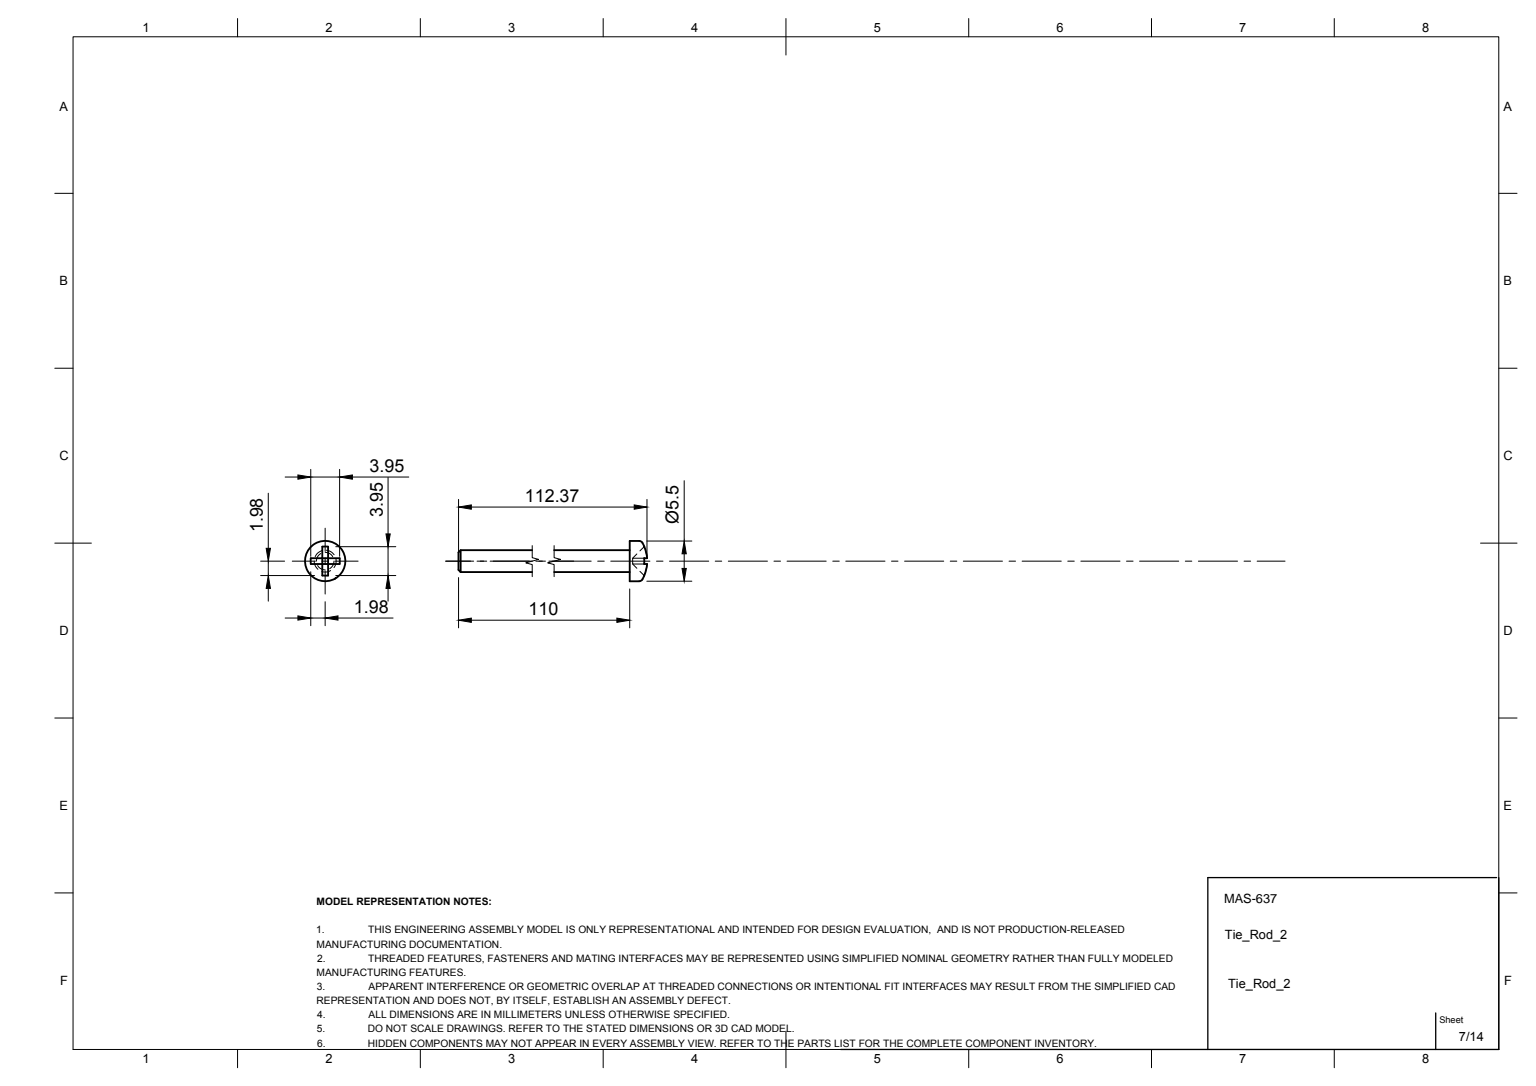
ISO-10303-21;
HEADER;
FILE_DESCRIPTION((''),'2;1');
FILE_NAME('Tie_Rod_2.step','2026-10-09T10:11:57-07:00',(''),(''),'','','');
FILE_SCHEMA (('AUTOMOTIVE_DESIGN { 1 0 10303 214 3 1 1 }'));
ENDSEC;
DATA;
#10=MECHANICAL_DESIGN_GEOMETRIC_PRESENTATION_REPRESENTATION('',(#127),#13510);
#72=SPHERICAL_SURFACE('',#8108,5.) ;
#97=SHAPE_REPRESENTATION_RELATIONSHIP('SRR','None',#13567,#112) ;
#112=ADVANCED_BREP_SHAPE_REPRESENTATION('',(#159),#13499) ;
#127=STYLED_ITEM('',(#13650),#159) ;
#159=MANIFOLD_SOLID_BREP('Body1',#7376) ;
#241=FACE_BOUND('',#1393,.T.) ;
#367=PLANE('',#8093) ;
#368=PLANE('',#8094) ;
#369=PLANE('',#8095) ;
#370=PLANE('',#8097) ;
#371=PLANE('',#8099) ;
#372=PLANE('',#8102) ;
#373=PLANE('',#8104) ;
#374=PLANE('',#8106) ;
#375=PLANE('',#8116) ;
#376=PLANE('',#8117) ;
#377=PLANE('',#8118) ;
#378=PLANE('',#8119) ;
#379=PLANE('',#8120) ;
#380=PLANE('',#8121) ;
#381=PLANE('',#8122) ;
#499=TOROIDAL_SURFACE('',#8082,2.25,0.5) ;
#634=CYLINDRICAL_SURFACE('',#8086,2.75) ;
#635=CYLINDRICAL_SURFACE('',#8088,1.5) ;
#886=FACE_OUTER_BOUND('',#1388,.T.) ;
#887=FACE_OUTER_BOUND('',#1389,.T.) ;
#888=FACE_OUTER_BOUND('',#1390,.T.) ;
#889=FACE_OUTER_BOUND('',#1391,.T.) ;
#890=FACE_OUTER_BOUND('',#1392,.T.) ;
#891=FACE_OUTER_BOUND('',#1394,.T.) ;
#892=FACE_OUTER_BOUND('',#1395,.T.) ;
#893=FACE_OUTER_BOUND('',#1396,.T.) ;
#894=FACE_OUTER_BOUND('',#1397,.T.) ;
#895=FACE_OUTER_BOUND('',#1398,.T.) ;
#896=FACE_OUTER_BOUND('',#1399,.T.) ;
#897=FACE_OUTER_BOUND('',#1400,.T.) ;
#898=FACE_OUTER_BOUND('',#1401,.T.) ;
#899=FACE_OUTER_BOUND('',#1402,.T.) ;
#900=FACE_OUTER_BOUND('',#1403,.T.) ;
#901=FACE_OUTER_BOUND('',#1404,.T.) ;
#902=FACE_OUTER_BOUND('',#1405,.T.) ;
#903=FACE_OUTER_BOUND('',#1406,.T.) ;
#904=FACE_OUTER_BOUND('',#1407,.T.) ;
#905=FACE_OUTER_BOUND('',#1408,.T.) ;
#1388=EDGE_LOOP('',(#5986,#5987,#5988,#5989)) ;
#1389=EDGE_LOOP('',(#5990,#5991,#5992,#5993)) ;
#1390=EDGE_LOOP('',(#5994,#5995,#5996,#5997)) ;
#1391=EDGE_LOOP('',(#5998,#5999,#6000,#6001)) ;
#1392=EDGE_LOOP('',(#6002)) ;
#1393=EDGE_LOOP('',(#6003)) ;
#1394=EDGE_LOOP('',(#6004)) ;
#1395=EDGE_LOOP('',(#6005,#6006,#6007,#6008)) ;
#1396=EDGE_LOOP('',(#6009,#6010,#6011,#6012)) ;
#1397=EDGE_LOOP('',(#6013,#6014,#6015,#6016)) ;
#1398=EDGE_LOOP('',(#6017,#6018,#6019)) ;
#1399=EDGE_LOOP('',(#6020,#6021,#6022)) ;
#1400=EDGE_LOOP('',(#6023,#6024,#6025)) ;
#1401=EDGE_LOOP('',(#6026,#6027,#6028,#6029,#6030,#6031,#6032,#6033,#6034,
#6035,#6036,#6037,#6038,#6039,#6040,#6041)) ;
#1402=EDGE_LOOP('',(#6042,#6043,#6044)) ;
#1403=EDGE_LOOP('',(#6045,#6046,#6047,#6048)) ;
#1404=EDGE_LOOP('',(#6049,#6050,#6051)) ;
#1405=EDGE_LOOP('',(#6052,#6053,#6054)) ;
#1406=EDGE_LOOP('',(#6055,#6056,#6057,#6058)) ;
#1407=EDGE_LOOP('',(#6059,#6060,#6061)) ;
#1408=EDGE_LOOP('',(#6062,#6063,#6064,#6065)) ;
#1925=LINE('',#12504,#2419) ;
#1926=LINE('',#12509,#2420) ;
#1927=LINE('',#12513,#2421) ;
#1928=LINE('',#12520,#2422) ;
#1929=LINE('',#12522,#2423) ;
#1930=LINE('',#12524,#2424) ;
#1931=LINE('',#12531,#2425) ;
#1932=LINE('',#12533,#2426) ;
#1933=LINE('',#12534,#2427) ;
#1934=LINE('',#12537,#2428) ;
#1935=LINE('',#12543,#2429) ;
#1936=LINE('',#12548,#2430) ;
#1937=LINE('',#12552,#2431) ;
#1938=LINE('',#12566,#2432) ;
#1939=LINE('',#12568,#2433) ;
#1940=LINE('',#12569,#2434) ;
#1941=LINE('',#12572,#2435) ;
#1942=LINE('',#12574,#2436) ;
#1943=LINE('',#12575,#2437) ;
#2419=VECTOR('',#9879,2.75) ;
#2420=VECTOR('',#9884,1.5) ;
#2421=VECTOR('',#9889,1.2) ;
#2422=VECTOR('',#9898,1.00000000000035) ;
#2423=VECTOR('',#9899,0.99999999999962) ;
#2424=VECTOR('',#9900,1.00000000000035) ;
#2425=VECTOR('',#9907,1.00000000000035) ;
#2426=VECTOR('',#9908,0.99999999999962) ;
#2427=VECTOR('',#9909,1.00000000000035) ;
#2428=VECTOR('',#9912,1.) ;
#2429=VECTOR('',#9919,1.) ;
#2430=VECTOR('',#9926,1.) ;
#2431=VECTOR('',#9931,1.) ;
#2432=VECTOR('',#9950,1.00000000000035) ;
#2433=VECTOR('',#9953,1.00000000000035) ;
#2434=VECTOR('',#9954,0.99999999999962) ;
#2435=VECTOR('',#9959,1.00000000000035) ;
#2436=VECTOR('',#9962,0.99999999999962) ;
#2437=VECTOR('',#9963,1.00000000000035) ;
#2919=CIRCLE('',#8083,2.75) ;
#2920=CIRCLE('',#8084,0.5) ;
#2921=CIRCLE('',#8085,2.5) ;
#2922=CIRCLE('',#8087,2.75) ;
#2923=CIRCLE('',#8089,1.5) ;
#2924=CIRCLE('',#8090,1.5) ;
#2925=CIRCLE('',#8092,1.2) ;
#2926=CIRCLE('',#8096,4.64997589841126) ;
#2927=CIRCLE('',#8098,4.64997589841224) ;
#2928=CIRCLE('',#8100,4.98397431775083) ;
#2929=CIRCLE('',#8101,4.98397431775083) ;
#2930=CIRCLE('',#8103,4.98396179815174) ;
#2931=CIRCLE('',#8105,4.98396179722269) ;
#2932=CIRCLE('',#8107,4.98397431775083) ;
#2933=CIRCLE('',#8109,5.) ;
#2934=CIRCLE('',#8110,4.9839743177514) ;
#2935=CIRCLE('',#8111,4.64973117502146) ;
#2936=CIRCLE('',#8112,4.9839743177522) ;
#2937=CIRCLE('',#8113,4.9839743177522) ;
#2938=CIRCLE('',#8114,4.64973117502146) ;
#2939=CIRCLE('',#8115,4.9839743177514) ;
#3519=VERTEX_POINT('',#12496) ;
#3520=VERTEX_POINT('',#12498) ;
#3521=VERTEX_POINT('',#12502) ;
#3522=VERTEX_POINT('',#12506) ;
#3523=VERTEX_POINT('',#12508) ;
#3524=VERTEX_POINT('',#12512) ;
#3525=VERTEX_POINT('',#12518) ;
#3526=VERTEX_POINT('',#12519) ;
#3527=VERTEX_POINT('',#12521) ;
#3528=VERTEX_POINT('',#12523) ;
#3529=VERTEX_POINT('',#12527) ;
#3530=VERTEX_POINT('',#12528) ;
#3531=VERTEX_POINT('',#12530) ;
#3532=VERTEX_POINT('',#12532) ;
#3533=VERTEX_POINT('',#12536) ;
#3534=VERTEX_POINT('',#12538) ;
#3535=VERTEX_POINT('',#12542) ;
#3536=VERTEX_POINT('',#12546) ;
#3537=VERTEX_POINT('',#12550) ;
#3538=VERTEX_POINT('',#12555) ;
#3539=VERTEX_POINT('',#12557) ;
#3540=VERTEX_POINT('',#12560) ;
#3541=VERTEX_POINT('',#12562) ;
#4380=EDGE_CURVE('',#3519,#3519,#2919,.T.) ;
#4381=EDGE_CURVE('',#3519,#3520,#2920,.T.) ;
#4382=EDGE_CURVE('',#3520,#3520,#2921,.T.) ;
#4383=EDGE_CURVE('',#3521,#3521,#2922,.T.) ;
#4384=EDGE_CURVE('',#3521,#3519,#1925,.T.) ;
#4385=EDGE_CURVE('',#3522,#3522,#2923,.T.) ;
#4386=EDGE_CURVE('',#3522,#3523,#1926,.T.) ;
#4387=EDGE_CURVE('',#3523,#3523,#2924,.T.) ;
#4388=EDGE_CURVE('',#3522,#3524,#1927,.T.) ;
#4389=EDGE_CURVE('',#3524,#3524,#2925,.F.) ;
#4390=EDGE_CURVE('',#3525,#3526,#1928,.T.) ;
#4391=EDGE_CURVE('',#3525,#3527,#1929,.F.) ;
#4392=EDGE_CURVE('',#3527,#3528,#1930,.T.) ;
#4393=EDGE_CURVE('',#3528,#3526,#2926,.T.) ;
#4394=EDGE_CURVE('',#3529,#3530,#2927,.T.) ;
#4395=EDGE_CURVE('',#3529,#3531,#1931,.F.) ;
#4396=EDGE_CURVE('',#3532,#3531,#1932,.F.) ;
#4397=EDGE_CURVE('',#3530,#3532,#1933,.F.) ;
#4398=EDGE_CURVE('',#3527,#3533,#1934,.T.) ;
#4399=EDGE_CURVE('',#3534,#3533,#2928,.F.) ;
#4400=EDGE_CURVE('',#3528,#3534,#2929,.F.) ;
#4401=EDGE_CURVE('',#3531,#3535,#1935,.T.) ;
#4402=EDGE_CURVE('',#3535,#3529,#2930,.T.) ;
#4403=EDGE_CURVE('',#3536,#3526,#2931,.T.) ;
#4404=EDGE_CURVE('',#3525,#3536,#1936,.T.) ;
#4405=EDGE_CURVE('',#3530,#3537,#2932,.F.) ;
#4406=EDGE_CURVE('',#3532,#3537,#1937,.T.) ;
#4407=EDGE_CURVE('',#3520,#3534,#2933,.T.) ;
#4408=EDGE_CURVE('',#3538,#3533,#2934,.T.) ;
#4409=EDGE_CURVE('',#3539,#3538,#2935,.T.) ;
#4410=EDGE_CURVE('',#3539,#3535,#2936,.T.) ;
#4411=EDGE_CURVE('',#3540,#3537,#2937,.T.) ;
#4412=EDGE_CURVE('',#3540,#3541,#2938,.T.) ;
#4413=EDGE_CURVE('',#3541,#3536,#2939,.T.) ;
#4414=EDGE_CURVE('',#3541,#3525,#1938,.F.) ;
#4415=EDGE_CURVE('',#3540,#3532,#1939,.F.) ;
#4416=EDGE_CURVE('',#3532,#3525,#1940,.T.) ;
#4417=EDGE_CURVE('',#3527,#3538,#1941,.T.) ;
#4418=EDGE_CURVE('',#3531,#3527,#1942,.T.) ;
#4419=EDGE_CURVE('',#3531,#3539,#1943,.T.) ;
#5986=ORIENTED_EDGE('',*,*,#4380,.F.) ;
#5987=ORIENTED_EDGE('',*,*,#4381,.T.) ;
#5988=ORIENTED_EDGE('',*,*,#4382,.T.) ;
#5989=ORIENTED_EDGE('',*,*,#4381,.F.) ;
#5990=ORIENTED_EDGE('',*,*,#4383,.F.) ;
#5991=ORIENTED_EDGE('',*,*,#4384,.T.) ;
#5992=ORIENTED_EDGE('',*,*,#4380,.T.) ;
#5993=ORIENTED_EDGE('',*,*,#4384,.F.) ;
#5994=ORIENTED_EDGE('',*,*,#4385,.F.) ;
#5995=ORIENTED_EDGE('',*,*,#4386,.T.) ;
#5996=ORIENTED_EDGE('',*,*,#4387,.T.) ;
#5997=ORIENTED_EDGE('',*,*,#4386,.F.) ;
#5998=ORIENTED_EDGE('',*,*,#4385,.T.) ;
#5999=ORIENTED_EDGE('',*,*,#4388,.T.) ;
#6000=ORIENTED_EDGE('',*,*,#4389,.F.) ;
#6001=ORIENTED_EDGE('',*,*,#4388,.F.) ;
#6002=ORIENTED_EDGE('',*,*,#4383,.T.) ;
#6003=ORIENTED_EDGE('',*,*,#4387,.F.) ;
#6004=ORIENTED_EDGE('',*,*,#4389,.T.) ;
#6005=ORIENTED_EDGE('',*,*,#4390,.F.) ;
#6006=ORIENTED_EDGE('',*,*,#4391,.T.) ;
#6007=ORIENTED_EDGE('',*,*,#4392,.T.) ;
#6008=ORIENTED_EDGE('',*,*,#4393,.T.) ;
#6009=ORIENTED_EDGE('',*,*,#4394,.F.) ;
#6010=ORIENTED_EDGE('',*,*,#4395,.T.) ;
#6011=ORIENTED_EDGE('',*,*,#4396,.F.) ;
#6012=ORIENTED_EDGE('',*,*,#4397,.F.) ;
#6013=ORIENTED_EDGE('',*,*,#4398,.T.) ;
#6014=ORIENTED_EDGE('',*,*,#4399,.F.) ;
#6015=ORIENTED_EDGE('',*,*,#4400,.F.) ;
#6016=ORIENTED_EDGE('',*,*,#4392,.F.) ;
#6017=ORIENTED_EDGE('',*,*,#4401,.F.) ;
#6018=ORIENTED_EDGE('',*,*,#4395,.F.) ;
#6019=ORIENTED_EDGE('',*,*,#4402,.F.) ;
#6020=ORIENTED_EDGE('',*,*,#4390,.T.) ;
#6021=ORIENTED_EDGE('',*,*,#4403,.F.) ;
#6022=ORIENTED_EDGE('',*,*,#4404,.F.) ;
#6023=ORIENTED_EDGE('',*,*,#4405,.F.) ;
#6024=ORIENTED_EDGE('',*,*,#4397,.T.) ;
#6025=ORIENTED_EDGE('',*,*,#4406,.T.) ;
#6026=ORIENTED_EDGE('',*,*,#4382,.F.) ;
#6027=ORIENTED_EDGE('',*,*,#4407,.T.) ;
#6028=ORIENTED_EDGE('',*,*,#4399,.T.) ;
#6029=ORIENTED_EDGE('',*,*,#4408,.F.) ;
#6030=ORIENTED_EDGE('',*,*,#4409,.F.) ;
#6031=ORIENTED_EDGE('',*,*,#4410,.T.) ;
#6032=ORIENTED_EDGE('',*,*,#4402,.T.) ;
#6033=ORIENTED_EDGE('',*,*,#4394,.T.) ;
#6034=ORIENTED_EDGE('',*,*,#4405,.T.) ;
#6035=ORIENTED_EDGE('',*,*,#4411,.F.) ;
#6036=ORIENTED_EDGE('',*,*,#4412,.T.) ;
#6037=ORIENTED_EDGE('',*,*,#4413,.T.) ;
#6038=ORIENTED_EDGE('',*,*,#4403,.T.) ;
#6039=ORIENTED_EDGE('',*,*,#4393,.F.) ;
#6040=ORIENTED_EDGE('',*,*,#4400,.T.) ;
#6041=ORIENTED_EDGE('',*,*,#4407,.F.) ;
#6042=ORIENTED_EDGE('',*,*,#4414,.T.) ;
#6043=ORIENTED_EDGE('',*,*,#4404,.T.) ;
#6044=ORIENTED_EDGE('',*,*,#4413,.F.) ;
#6045=ORIENTED_EDGE('',*,*,#4414,.F.) ;
#6046=ORIENTED_EDGE('',*,*,#4412,.F.) ;
#6047=ORIENTED_EDGE('',*,*,#4415,.T.) ;
#6048=ORIENTED_EDGE('',*,*,#4416,.T.) ;
#6049=ORIENTED_EDGE('',*,*,#4411,.T.) ;
#6050=ORIENTED_EDGE('',*,*,#4406,.F.) ;
#6051=ORIENTED_EDGE('',*,*,#4415,.F.) ;
#6052=ORIENTED_EDGE('',*,*,#4417,.T.) ;
#6053=ORIENTED_EDGE('',*,*,#4408,.T.) ;
#6054=ORIENTED_EDGE('',*,*,#4398,.F.) ;
#6055=ORIENTED_EDGE('',*,*,#4417,.F.) ;
#6056=ORIENTED_EDGE('',*,*,#4418,.F.) ;
#6057=ORIENTED_EDGE('',*,*,#4419,.T.) ;
#6058=ORIENTED_EDGE('',*,*,#4409,.T.) ;
#6059=ORIENTED_EDGE('',*,*,#4401,.T.) ;
#6060=ORIENTED_EDGE('',*,*,#4410,.F.) ;
#6061=ORIENTED_EDGE('',*,*,#4419,.F.) ;
#6062=ORIENTED_EDGE('',*,*,#4418,.T.) ;
#6063=ORIENTED_EDGE('',*,*,#4391,.F.) ;
#6064=ORIENTED_EDGE('',*,*,#4416,.F.) ;
#6065=ORIENTED_EDGE('',*,*,#4396,.T.) ;
#6886=CONICAL_SURFACE('',#8091,1.2,0.785398163397) ;
#7136=ADVANCED_FACE('',(#886),#499,.T.) ;
#7137=ADVANCED_FACE('',(#887),#634,.T.) ;
#7138=ADVANCED_FACE('',(#888),#635,.T.) ;
#7139=ADVANCED_FACE('',(#889),#6886,.T.) ;
#7140=ADVANCED_FACE('',(#890,#241),#367,.T.) ;
#7141=ADVANCED_FACE('',(#891),#368,.T.) ;
#7142=ADVANCED_FACE('',(#892),#369,.T.) ;
#7143=ADVANCED_FACE('',(#893),#370,.F.) ;
#7144=ADVANCED_FACE('',(#894),#371,.F.) ;
#7145=ADVANCED_FACE('',(#895),#372,.F.) ;
#7146=ADVANCED_FACE('',(#896),#373,.T.) ;
#7147=ADVANCED_FACE('',(#897),#374,.T.) ;
#7148=ADVANCED_FACE('',(#898),#72,.T.) ;
#7149=ADVANCED_FACE('',(#899),#375,.T.) ;
#7150=ADVANCED_FACE('',(#900),#376,.F.) ;
#7151=ADVANCED_FACE('',(#901),#377,.F.) ;
#7152=ADVANCED_FACE('',(#902),#378,.T.) ;
#7153=ADVANCED_FACE('',(#903),#379,.T.) ;
#7154=ADVANCED_FACE('',(#904),#380,.F.) ;
#7155=ADVANCED_FACE('',(#905),#381,.F.) ;
#7376=CLOSED_SHELL('',(#7136,#7137,#7138,#7139,#7140,#7141,#7142,#7143,
#7144,#7145,#7146,#7147,#7148,#7149,#7150,#7151,#7152,#7153,#7154,#7155)) ;
#8081=AXIS2_PLACEMENT_3D('',#12494,#9865,#9866) ;
#8082=AXIS2_PLACEMENT_3D('',#12495,#9867,#9868) ;
#8083=AXIS2_PLACEMENT_3D('',#12497,#9869,#9870) ;
#8084=AXIS2_PLACEMENT_3D('',#12499,#9871,#9872) ;
#8085=AXIS2_PLACEMENT_3D('',#12500,#9873,#9874) ;
#8086=AXIS2_PLACEMENT_3D('',#12501,#9875,#9876) ;
#8087=AXIS2_PLACEMENT_3D('',#12503,#9877,#9878) ;
#8088=AXIS2_PLACEMENT_3D('',#12505,#9880,#9881) ;
#8089=AXIS2_PLACEMENT_3D('',#12507,#9882,#9883) ;
#8090=AXIS2_PLACEMENT_3D('',#12510,#9885,#9886) ;
#8091=AXIS2_PLACEMENT_3D('',#12511,#9887,#9888) ;
#8092=AXIS2_PLACEMENT_3D('',#12514,#9890,#9891) ;
#8093=AXIS2_PLACEMENT_3D('',#12515,#9892,#9893) ;
#8094=AXIS2_PLACEMENT_3D('',#12516,#9894,#9895) ;
#8095=AXIS2_PLACEMENT_3D('',#12517,#9896,#9897) ;
#8096=AXIS2_PLACEMENT_3D('',#12525,#9901,#9902) ;
#8097=AXIS2_PLACEMENT_3D('',#12526,#9903,#9904) ;
#8098=AXIS2_PLACEMENT_3D('',#12529,#9905,#9906) ;
#8099=AXIS2_PLACEMENT_3D('',#12535,#9910,#9911) ;
#8100=AXIS2_PLACEMENT_3D('',#12539,#9913,#9914) ;
#8101=AXIS2_PLACEMENT_3D('',#12540,#9915,#9916) ;
#8102=AXIS2_PLACEMENT_3D('',#12541,#9917,#9918) ;
#8103=AXIS2_PLACEMENT_3D('',#12544,#9920,#9921) ;
#8104=AXIS2_PLACEMENT_3D('',#12545,#9922,#9923) ;
#8105=AXIS2_PLACEMENT_3D('',#12547,#9924,#9925) ;
#8106=AXIS2_PLACEMENT_3D('',#12549,#9927,#9928) ;
#8107=AXIS2_PLACEMENT_3D('',#12551,#9929,#9930) ;
#8108=AXIS2_PLACEMENT_3D('',#12553,#9932,#9933) ;
#8109=AXIS2_PLACEMENT_3D('',#12554,#9934,#9935) ;
#8110=AXIS2_PLACEMENT_3D('',#12556,#9936,#9937) ;
#8111=AXIS2_PLACEMENT_3D('',#12558,#9938,#9939) ;
#8112=AXIS2_PLACEMENT_3D('',#12559,#9940,#9941) ;
#8113=AXIS2_PLACEMENT_3D('',#12561,#9942,#9943) ;
#8114=AXIS2_PLACEMENT_3D('',#12563,#9944,#9945) ;
#8115=AXIS2_PLACEMENT_3D('',#12564,#9946,#9947) ;
#8116=AXIS2_PLACEMENT_3D('',#12565,#9948,#9949) ;
#8117=AXIS2_PLACEMENT_3D('',#12567,#9951,#9952) ;
#8118=AXIS2_PLACEMENT_3D('',#12570,#9955,#9956) ;
#8119=AXIS2_PLACEMENT_3D('',#12571,#9957,#9958) ;
#8120=AXIS2_PLACEMENT_3D('',#12573,#9960,#9961) ;
#8121=AXIS2_PLACEMENT_3D('',#12576,#9964,#9965) ;
#8122=AXIS2_PLACEMENT_3D('',#12577,#9966,#9967) ;
#9865=DIRECTION('axis',(0.,0.,1.)) ;
#9866=DIRECTION('refdir',(1.,0.,0.)) ;
#9867=DIRECTION('center_axis',(0.,0.,1.)) ;
#9868=DIRECTION('ref_axis',(-0.520296023213257,-0.853985976599423,0.)) ;
#9869=DIRECTION('center_axis',(0.,0.,1.)) ;
#9870=DIRECTION('ref_axis',(-1.,0.,0.)) ;
#9871=DIRECTION('center_axis',(-0.853985976599423,0.520296023213257,0.)) ;
#9872=DIRECTION('ref_axis',(0.520296023213257,0.853985976599423,0.)) ;
#9873=DIRECTION('center_axis',(0.,0.,1.)) ;
#9874=DIRECTION('ref_axis',(-1.,0.,0.)) ;
#9875=DIRECTION('center_axis',(0.,0.,1.)) ;
#9876=DIRECTION('ref_axis',(-0.520296023213258,-0.853985976599422,0.)) ;
#9877=DIRECTION('center_axis',(0.,0.,1.)) ;
#9878=DIRECTION('ref_axis',(-1.,0.,0.)) ;
#9879=DIRECTION('',(0.,0.,-1.)) ;
#9880=DIRECTION('center_axis',(0.,0.,1.)) ;
#9881=DIRECTION('ref_axis',(-0.520296023213257,-0.853985976599423,0.)) ;
#9882=DIRECTION('center_axis',(0.,0.,1.)) ;
#9883=DIRECTION('ref_axis',(-1.,0.,0.)) ;
#9884=DIRECTION('',(0.,0.,-1.)) ;
#9885=DIRECTION('center_axis',(0.,0.,1.)) ;
#9886=DIRECTION('ref_axis',(-1.,0.,0.)) ;
#9887=DIRECTION('center_axis',(0.,0.,-1.)) ;
#9888=DIRECTION('ref_axis',(-0.520296023213257,-0.853985976599423,0.)) ;
#9889=DIRECTION('',(-0.367904846238322,-0.603859275091397,0.707106781186864)) ;
#9890=DIRECTION('center_axis',(0.,0.,-1.)) ;
#9891=DIRECTION('ref_axis',(1.,0.,0.)) ;
#9892=DIRECTION('center_axis',(0.,0.,1.)) ;
#9893=DIRECTION('ref_axis',(1.,0.,0.)) ;
#9894=DIRECTION('center_axis',(0.,0.,1.)) ;
#9895=DIRECTION('ref_axis',(1.,0.,0.)) ;
#9896=DIRECTION('center_axis',(-0.612372435695786,-0.353553390592877,-0.707106781186753)) ;
#9897=DIRECTION('ref_axis',(0.612372435696143,0.353553390593082,-0.707106781186342)) ;
#9898=DIRECTION('',(0.612372435695786,0.353553390592877,-0.707106781186753)) ;
#9899=DIRECTION('',(0.50000000000019,-0.866025403784329,0.)) ;
#9900=DIRECTION('',(0.612372435695786,0.353553390592877,-0.707106781186753)) ;
#9901=DIRECTION('center_axis',(-0.612372436109239,-0.353553390846033,-0.707106780702115)) ;
#9902=DIRECTION('ref_axis',(0.653113494420765,0.277745658422985,-0.704485707898095)) ;
#9903=DIRECTION('center_axis',(-0.612372435695786,-0.353553390592877,0.707106781186753)) ;
#9904=DIRECTION('ref_axis',(-0.612372435696143,-0.353553390593082,-0.707106781186342)) ;
#9905=DIRECTION('center_axis',(-0.612372436109373,-0.35355339084611,0.70710678070196)) ;
#9906=DIRECTION('ref_axis',(-0.567091543180707,-0.426740048530749,-0.70448570789825)) ;
#9907=DIRECTION('',(-0.612372435695786,-0.353553390592877,-0.707106781186753)) ;
#9908=DIRECTION('',(0.50000000000019,-0.866025403784329,0.)) ;
#9909=DIRECTION('',(-0.612372435695786,-0.353553390592877,-0.707106781186753)) ;
#9910=DIRECTION('center_axis',(-0.50000000000019,0.866025403784329,0.)) ;
#9911=DIRECTION('ref_axis',(-0.866025403784329,-0.50000000000019,0.)) ;
#9912=DIRECTION('',(0.,0.,-1.)) ;
#9913=DIRECTION('center_axis',(0.50000000000019,-0.866025403784329,0.)) ;
#9914=DIRECTION('ref_axis',(0.,0.,-1.)) ;
#9915=DIRECTION('center_axis',(0.50000000000019,-0.866025403784329,0.)) ;
#9916=DIRECTION('ref_axis',(0.,0.,-1.)) ;
#9917=DIRECTION('center_axis',(-0.50000000000019,0.866025403784329,0.)) ;
#9918=DIRECTION('ref_axis',(-0.866025403784329,-0.50000000000019,0.)) ;
#9919=DIRECTION('',(0.,0.,-1.)) ;
#9920=DIRECTION('center_axis',(-0.500000000086009,0.866025403734781,-4.5051562602977E-10)) ;
#9921=DIRECTION('ref_axis',(-0.343296529291604,-0.198202344121424,-0.91807588126533)) ;
#9922=DIRECTION('center_axis',(-0.50000000000019,0.866025403784329,0.)) ;
#9923=DIRECTION('ref_axis',(-0.866025403784329,-0.50000000000019,0.)) ;
#9924=DIRECTION('center_axis',(0.500000000055529,-0.866025403752379,-1.8165075282686E-10)) ;
#9925=DIRECTION('ref_axis',(0.343296529449915,0.198202343911691,-0.918075881251411)) ;
#9926=DIRECTION('',(0.,0.,-1.)) ;
#9927=DIRECTION('center_axis',(-0.50000000000019,0.866025403784329,0.)) ;
#9928=DIRECTION('ref_axis',(-0.866025403784329,-0.50000000000019,0.)) ;
#9929=DIRECTION('center_axis',(-0.50000000000019,0.866025403784329,0.)) ;
#9930=DIRECTION('ref_axis',(0.,0.,-1.)) ;
#9931=DIRECTION('',(0.,0.,-1.)) ;
#9932=DIRECTION('center_axis',(0.,0.,1.)) ;
#9933=DIRECTION('ref_axis',(-0.520296023213258,-0.853985976599422,0.)) ;
#9934=DIRECTION('center_axis',(-0.853985976599422,0.520296023213258,0.)) ;
#9935=DIRECTION('ref_axis',(0.520296023213258,0.853985976599422,0.)) ;
#9936=DIRECTION('center_axis',(-0.866025403784329,-0.50000000000019,0.)) ;
#9937=DIRECTION('ref_axis',(0.,0.,1.)) ;
#9938=DIRECTION('center_axis',(0.353553390592877,-0.612372435695786,-0.707106781186753)) ;
#9939=DIRECTION('ref_axis',(-1.27819621364487E-16,-0.755928946018553,0.654653670707863)) ;
#9940=DIRECTION('center_axis',(-0.866025403784329,-0.50000000000019,0.)) ;
#9941=DIRECTION('ref_axis',(0.,0.,1.)) ;
#9942=DIRECTION('center_axis',(0.866025403784329,0.50000000000019,0.)) ;
#9943=DIRECTION('ref_axis',(0.,0.,1.)) ;
#9944=DIRECTION('center_axis',(0.353553390592877,-0.612372435695786,0.707106781186753)) ;
#9945=DIRECTION('ref_axis',(1.27819621364487E-16,0.755928946018553,0.654653670707863)) ;
#9946=DIRECTION('center_axis',(0.866025403784329,0.50000000000019,0.)) ;
#9947=DIRECTION('ref_axis',(0.,0.,1.)) ;
#9948=DIRECTION('center_axis',(-0.866025403784329,-0.50000000000019,0.)) ;
#9949=DIRECTION('ref_axis',(0.50000000000019,-0.866025403784329,0.)) ;
#9950=DIRECTION('',(0.353553390592877,-0.612372435695786,-0.707106781186753)) ;
#9951=DIRECTION('center_axis',(0.353553390592877,-0.612372435695786,0.707106781186753)) ;
#9952=DIRECTION('ref_axis',(0.353553390593082,-0.612372435696143,-0.707106781186342)) ;
#9953=DIRECTION('',(0.353553390592877,-0.612372435695786,-0.707106781186753)) ;
#9954=DIRECTION('',(0.866025403784329,0.50000000000019,0.)) ;
#9955=DIRECTION('center_axis',(-0.866025403784329,-0.50000000000019,0.)) ;
#9956=DIRECTION('ref_axis',(0.50000000000019,-0.866025403784329,0.)) ;
#9957=DIRECTION('center_axis',(-0.866025403784329,-0.50000000000019,0.)) ;
#9958=DIRECTION('ref_axis',(0.50000000000019,-0.866025403784329,0.)) ;
#9959=DIRECTION('',(-0.353553390592877,0.612372435695786,-0.707106781186753)) ;
#9960=DIRECTION('center_axis',(0.353553390592877,-0.612372435695786,-0.707106781186753)) ;
#9961=DIRECTION('ref_axis',(-0.353553390593082,0.612372435696143,-0.707106781186342)) ;
#9962=DIRECTION('',(0.866025403784329,0.50000000000019,0.)) ;
#9963=DIRECTION('',(-0.353553390592877,0.612372435695786,-0.707106781186753)) ;
#9964=DIRECTION('center_axis',(-0.866025403784329,-0.50000000000019,0.)) ;
#9965=DIRECTION('ref_axis',(0.50000000000019,-0.866025403784329,0.)) ;
#9966=DIRECTION('center_axis',(0.,0.,1.)) ;
#9967=DIRECTION('ref_axis',(0.,1.,0.)) ;
#12494=CARTESIAN_POINT('',(0.,0.,0.)) ;
#12495=CARTESIAN_POINT('Origin',(-21.6506350946,-12.5,7.50288568297)) ;
#12496=CARTESIAN_POINT('',(-20.2198210307635,-10.1515385643516,7.50288568297)) ;
#12497=CARTESIAN_POINT('Origin',(-21.6506350946,-12.5,7.50288568297)) ;
#12498=CARTESIAN_POINT('',(-20.3498950365669,-10.3650350585014,7.06987298108)) ;
#12499=CARTESIAN_POINT('Origin',(-20.4799690423702,-10.5785315526513,7.50288568297)) ;
#12500=CARTESIAN_POINT('Origin',(-21.6506350946,-12.5,7.06987298108)) ;
#12501=CARTESIAN_POINT('Origin',(-21.6506350946,-12.5,62.6)) ;
#12502=CARTESIAN_POINT('',(-20.2198210307635,-10.1515385643516,8.8)) ;
#12503=CARTESIAN_POINT('Origin',(-21.6506350946,-12.5,8.8)) ;
#12504=CARTESIAN_POINT('',(-20.2198210307635,-10.1515385643516,62.6)) ;
#12505=CARTESIAN_POINT('Origin',(-21.6506350946,-12.5,62.6)) ;
#12506=CARTESIAN_POINT('',(-20.8701910597801,-11.2190210351009,118.5)) ;
#12507=CARTESIAN_POINT('Origin',(-21.6506350946,-12.5,118.5)) ;
#12508=CARTESIAN_POINT('',(-20.8701910597801,-11.2190210351009,8.8)) ;
#12509=CARTESIAN_POINT('',(-20.8701910597801,-11.2190210351009,62.6)) ;
#12510=CARTESIAN_POINT('Origin',(-21.6506350946,-12.5,8.8)) ;
#12511=CARTESIAN_POINT('Origin',(-21.6506350946,-12.5,118.8)) ;
#12512=CARTESIAN_POINT('',(-21.0262798667441,-11.4752168280807,118.8)) ;
#12513=CARTESIAN_POINT('',(-21.0262798667441,-11.4752168280807,118.8)) ;
#12514=CARTESIAN_POINT('Origin',(-21.6506350946,-12.5,118.8)) ;
#12515=CARTESIAN_POINT('Origin',(0.,26.5,8.8)) ;
#12516=CARTESIAN_POINT('Origin',(0.,25.,118.8)) ;
#12517=CARTESIAN_POINT('Origin',(-21.3042249331,-12.3,8.4)) ;
#12518=CARTESIAN_POINT('',(-21.1042249331,-12.6464101615,8.4)) ;
#12519=CARTESIAN_POINT('',(-19.7396566270596,-11.8585762927655,6.82433230688143)) ;
#12520=CARTESIAN_POINT('',(-20.4219407311,-12.2524931938,7.61216606458)) ;
#12521=CARTESIAN_POINT('',(-21.5042249331,-11.9535898385,8.4)) ;
#12522=CARTESIAN_POINT('',(-21.2042249331,-12.4732050808,8.4)) ;
#12523=CARTESIAN_POINT('',(-20.139656529,-11.1657559031,6.82433212917)) ;
#12524=CARTESIAN_POINT('',(-20.8219407311,-11.5596728708,7.61216606458)) ;
#12525=CARTESIAN_POINT('Origin',(-22.7766185369837,-13.1500868436552,10.1001736916713)) ;
#12526=CARTESIAN_POINT('Origin',(-21.9970452561,-12.7,8.4)) ;
#12527=CARTESIAN_POINT('',(-23.5616135621925,-13.1414237072081,6.82433230688583)) ;
#12528=CARTESIAN_POINT('',(-23.1616136602,-13.8342440969,6.82433212917)) ;
#12529=CARTESIAN_POINT('Origin',(-20.5246516522163,-11.8499131563447,10.1001736916727)) ;
#12530=CARTESIAN_POINT('',(-22.1970452561,-12.3535898385,8.4)) ;
#12531=CARTESIAN_POINT('',(-22.8793294582,-12.7475068062,7.61216606458)) ;
#12532=CARTESIAN_POINT('',(-21.7970452561,-13.0464101615,8.4)) ;
#12533=CARTESIAN_POINT('',(-22.0970452561,-12.5267949192,8.4)) ;
#12534=CARTESIAN_POINT('',(-22.4793294582,-13.4403271292,7.61216606458)) ;
#12535=CARTESIAN_POINT('Origin',(-0.2,0.346410161514,0.)) ;
#12536=CARTESIAN_POINT('',(-21.5042249330181,-11.9535898381328,6.43210306118512)) ;
#12537=CARTESIAN_POINT('',(-21.5042249331,-11.9535898385,7.41605197605)) ;
#12538=CARTESIAN_POINT('',(-21.2165355472721,-11.787492294143,6.47010239943018)) ;
#12539=CARTESIAN_POINT('Origin',(-21.8506350946002,-12.1535898384861,11.4)) ;
#12540=CARTESIAN_POINT('Origin',(-21.8506350946002,-12.1535898384861,11.4)) ;
#12541=CARTESIAN_POINT('Origin',(-0.2,0.346410161514,0.)) ;
#12542=CARTESIAN_POINT('',(-22.1970452563,-12.3535898385438,6.43210306142835)) ;
#12543=CARTESIAN_POINT('',(-22.1970452561,-12.3535898385,7.41605153106)) ;
#12544=CARTESIAN_POINT('Origin',(-21.8506365863726,-12.1535906970947,11.3999875799409)) ;
#12545=CARTESIAN_POINT('Origin',(0.2,-0.346410161514,0.)) ;
#12546=CARTESIAN_POINT('',(-21.1042249328953,-12.6464101614534,6.43210306142902)) ;
#12547=CARTESIAN_POINT('Origin',(-21.4506336033975,-12.8464093016759,11.3999875790186)) ;
#12548=CARTESIAN_POINT('',(-21.1042249331,-12.6464101615,7.41605153106)) ;
#12549=CARTESIAN_POINT('Origin',(0.2,-0.346410161514,0.)) ;
#12550=CARTESIAN_POINT('',(-21.7970452561761,-13.0464101618639,6.43210306118433)) ;
#12551=CARTESIAN_POINT('Origin',(-21.4506350945998,-12.8464101615139,11.4)) ;
#12552=CARTESIAN_POINT('',(-21.7970452561,-13.0464101615,7.41605197605)) ;
#12553=CARTESIAN_POINT('Origin',(-21.6506350946,-12.5,11.4)) ;
#12554=CARTESIAN_POINT('Origin',(-21.6506350946,-12.5,11.4)) ;
#12555=CARTESIAN_POINT('',(-22.2920588685,-10.5890214344,6.82433212917)) ;
#12556=CARTESIAN_POINT('Origin',(-21.3042249330923,-12.3000000000034,11.4)) ;
#12557=CARTESIAN_POINT('',(-22.9848791913296,-10.9890214349269,6.82433212927477)) ;
#12558=CARTESIAN_POINT('Origin',(-21.0006350945975,-13.6258330249253,10.0999999999932)) ;
#12559=CARTESIAN_POINT('Origin',(-21.9970452560991,-12.6999999999916,11.4)) ;
#12560=CARTESIAN_POINT('',(-21.0092113210215,-14.4109785651489,6.82433212927709)) ;
#12561=CARTESIAN_POINT('Origin',(-21.9970452560991,-12.6999999999916,11.4)) ;
#12562=CARTESIAN_POINT('',(-20.3163909977,-14.0109785656,6.82433212917)) ;
#12563=CARTESIAN_POINT('Origin',(-22.3006350946025,-11.3741669750747,10.0999999999932)) ;
#12564=CARTESIAN_POINT('Origin',(-21.3042249330923,-12.3000000000034,11.4)) ;
#12565=CARTESIAN_POINT('Origin',(-33.8042249331,9.35063509461,0.)) ;
#12566=CARTESIAN_POINT('',(-20.7103079654,-13.3286943635,7.61216606458)) ;
#12567=CARTESIAN_POINT('Origin',(-21.4506350946,-12.8464101615,8.4)) ;
#12568=CARTESIAN_POINT('',(-21.4031283511,-13.7286942549,7.61216619003)) ;
#12569=CARTESIAN_POINT('',(-21.6238401754,-12.9464101615,8.4)) ;
#12570=CARTESIAN_POINT('Origin',(-34.4970452561,8.95063509461,0.)) ;
#12571=CARTESIAN_POINT('Origin',(-33.8042249331,9.35063509461,0.)) ;
#12572=CARTESIAN_POINT('',(-21.8981419008,-11.2713056365,7.61216606458)) ;
#12573=CARTESIAN_POINT('Origin',(-21.8506350946,-12.1535898385,8.4)) ;
#12574=CARTESIAN_POINT('',(-21.6774300139,-12.0535898385,8.4)) ;
#12575=CARTESIAN_POINT('',(-22.5909621611,-11.6713057451,7.61216619003)) ;
#12576=CARTESIAN_POINT('Origin',(-34.4970452561,8.95063509461,0.)) ;
#12577=CARTESIAN_POINT('Origin',(0.,24.6,8.4)) ;
#13482=UNCERTAINTY_MEASURE_WITH_UNIT(LENGTH_MEASURE(0.01),#13511,
'DISTANCE_ACCURACY_VALUE',
'Maximum model space distance between geometric entities at asserted c
onnectivities') ;
#13493=UNCERTAINTY_MEASURE_WITH_UNIT(LENGTH_MEASURE(0.01),#13511,
'DISTANCE_ACCURACY_VALUE',
'Maximum model space distance between geometric entities at asserted c
onnectivities') ;
#13499=(
GEOMETRIC_REPRESENTATION_CONTEXT(3)
GLOBAL_UNCERTAINTY_ASSIGNED_CONTEXT((#13482))
GLOBAL_UNIT_ASSIGNED_CONTEXT((#13511,#13513,#13514))
REPRESENTATION_CONTEXT('','3D')
) ;
#13510=(
GEOMETRIC_REPRESENTATION_CONTEXT(3)
GLOBAL_UNCERTAINTY_ASSIGNED_CONTEXT((#13493))
GLOBAL_UNIT_ASSIGNED_CONTEXT((#13511,#13513,#13514))
REPRESENTATION_CONTEXT('','3D')
) ;
#13511=(
LENGTH_UNIT()
NAMED_UNIT(*)
SI_UNIT(.MILLI.,.METRE.)
) ;
#13513=(
NAMED_UNIT(*)
PLANE_ANGLE_UNIT()
SI_UNIT($,.RADIAN.)
) ;
#13514=(
NAMED_UNIT(*)
SI_UNIT($,.STERADIAN.)
SOLID_ANGLE_UNIT()
) ;
#13520=SHAPE_DEFINITION_REPRESENTATION(#13536,#13567) ;
#13536=PRODUCT_DEFINITION_SHAPE('',$,#13584) ;
#13567=SHAPE_REPRESENTATION('',(#8081),#13499) ;
#13578=PRODUCT_DEFINITION_CONTEXT('part definition',#13628,'design') ;
#13584=PRODUCT_DEFINITION('Tie_Rod_2','Tie_Rod_2',#13600,#13578) ;
#13600=PRODUCT_DEFINITION_FORMATION('',$,#13635) ;
#13628=APPLICATION_CONTEXT(
'Core Data for Automotive Mechanical Design Process') ;
#13629=PRODUCT_CONTEXT('part definition',#13628,'mechanical') ;
#13635=PRODUCT('Tie_Rod_2','Tie_Rod_2',$,(#13629)) ;
#13650=PRESENTATION_STYLE_ASSIGNMENT((#13655)) ;
#13655=SURFACE_STYLE_USAGE(.BOTH.,#13660) ;
#13660=SURFACE_SIDE_STYLE('',(#13665)) ;
#13665=SURFACE_STYLE_FILL_AREA(#13670) ;
#13670=FILL_AREA_STYLE('Opaque(144,144,144)',(#13675)) ;
#13675=FILL_AREA_STYLE_COLOUR('Opaque(144,144,144)',#13680) ;
#13680=COLOUR_RGB('Opaque(144,144,144)', 0.40784314, 0.44705882, 0.49803922) ;
ENDSEC;
END-ISO-10303-21;
